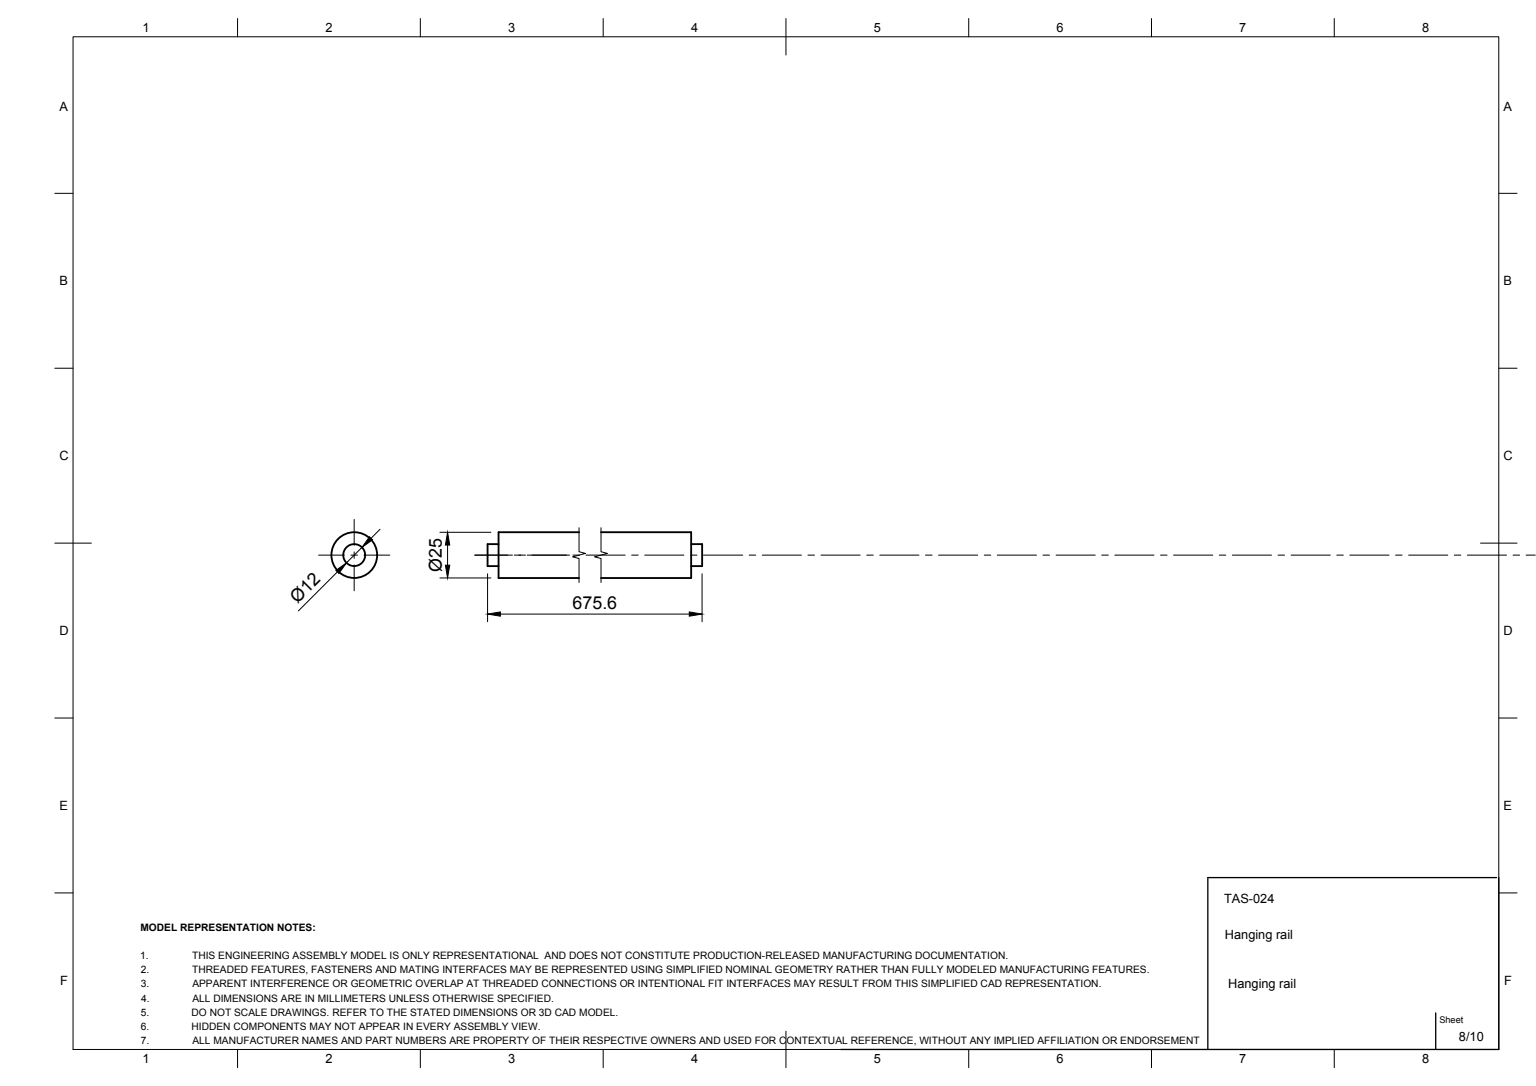
ISO-10303-21;
HEADER;
/* Generated by software containing ST-Developer
 * from STEP Tools, Inc. (www.steptools.com) 
 */

FILE_DESCRIPTION(
/* description */ (''),
/* implementation_level */ '2;1');

FILE_NAME(
/* name */ 'Hanging rail.step',
/* time_stamp */ '2026-11-15T17:53:25-08:00',
/* author */ (''),
/* organization */ (''),
/* preprocessor_version */ 'ST-DEVELOPER v20.2',
/* originating_system */ 'Autodesk Translation Framework v15.17.0.0',
/* authorisation */ '');

FILE_SCHEMA (('AUTOMOTIVE_DESIGN { 1 0 10303 214 3 1 1 }'));
ENDSEC;

DATA;
#10=MECHANICAL_DESIGN_GEOMETRIC_PRESENTATION_REPRESENTATION('',(#136),#2673);
#120=SHAPE_REPRESENTATION_RELATIONSHIP('SRR','None',#2728,#128);
#128=ADVANCED_BREP_SHAPE_REPRESENTATION('',(#144),#2670);
#136=STYLED_ITEM('',(#2777),#144);
#144=MANIFOLD_SOLID_BREP('Body1',#1522);
#157=FACE_BOUND('',#412,.T.);
#158=FACE_BOUND('',#414,.T.);
#224=PLANE('',#1718);
#225=PLANE('',#1722);
#226=PLANE('',#1726);
#227=PLANE('',#1727);
#307=FACE_OUTER_BOUND('',#406,.T.);
#308=FACE_OUTER_BOUND('',#407,.T.);
#309=FACE_OUTER_BOUND('',#408,.T.);
#310=FACE_OUTER_BOUND('',#409,.T.);
#311=FACE_OUTER_BOUND('',#410,.T.);
#312=FACE_OUTER_BOUND('',#411,.T.);
#313=FACE_OUTER_BOUND('',#413,.T.);
#406=EDGE_LOOP('',(#1376,#1377,#1378,#1379));
#407=EDGE_LOOP('',(#1380));
#408=EDGE_LOOP('',(#1381,#1382,#1383,#1384));
#409=EDGE_LOOP('',(#1385));
#410=EDGE_LOOP('',(#1386,#1387,#1388,#1389));
#411=EDGE_LOOP('',(#1390));
#412=EDGE_LOOP('',(#1391));
#413=EDGE_LOOP('',(#1392));
#414=EDGE_LOOP('',(#1393));
#566=LINE('',#2585,#714);
#567=LINE('',#2592,#715);
#568=LINE('',#2599,#716);
#714=VECTOR('',#2118,0.6);
#715=VECTOR('',#2127,0.6);
#716=VECTOR('',#2136,1.25);
#740=CIRCLE('',#1716,0.6);
#741=CIRCLE('',#1717,0.6);
#742=CIRCLE('',#1720,0.6);
#743=CIRCLE('',#1721,0.6);
#744=CIRCLE('',#1724,1.25);
#745=CIRCLE('',#1725,1.25);
#860=VERTEX_POINT('',#2582);
#861=VERTEX_POINT('',#2584);
#862=VERTEX_POINT('',#2589);
#863=VERTEX_POINT('',#2591);
#864=VERTEX_POINT('',#2596);
#865=VERTEX_POINT('',#2598);
#1034=EDGE_CURVE('',#860,#860,#740,.T.);
#1035=EDGE_CURVE('',#860,#861,#566,.T.);
#1036=EDGE_CURVE('',#861,#861,#741,.T.);
#1037=EDGE_CURVE('',#862,#862,#742,.T.);
#1038=EDGE_CURVE('',#862,#863,#567,.T.);
#1039=EDGE_CURVE('',#863,#863,#743,.T.);
#1040=EDGE_CURVE('',#864,#864,#744,.T.);
#1041=EDGE_CURVE('',#864,#865,#568,.T.);
#1042=EDGE_CURVE('',#865,#865,#745,.T.);
#1376=ORIENTED_EDGE('',*,*,#1034,.F.);
#1377=ORIENTED_EDGE('',*,*,#1035,.T.);
#1378=ORIENTED_EDGE('',*,*,#1036,.F.);
#1379=ORIENTED_EDGE('',*,*,#1035,.F.);
#1380=ORIENTED_EDGE('',*,*,#1034,.T.);
#1381=ORIENTED_EDGE('',*,*,#1037,.F.);
#1382=ORIENTED_EDGE('',*,*,#1038,.T.);
#1383=ORIENTED_EDGE('',*,*,#1039,.T.);
#1384=ORIENTED_EDGE('',*,*,#1038,.F.);
#1385=ORIENTED_EDGE('',*,*,#1039,.F.);
#1386=ORIENTED_EDGE('',*,*,#1040,.F.);
#1387=ORIENTED_EDGE('',*,*,#1041,.T.);
#1388=ORIENTED_EDGE('',*,*,#1042,.T.);
#1389=ORIENTED_EDGE('',*,*,#1041,.F.);
#1390=ORIENTED_EDGE('',*,*,#1040,.T.);
#1391=ORIENTED_EDGE('',*,*,#1036,.T.);
#1392=ORIENTED_EDGE('',*,*,#1042,.F.);
#1393=ORIENTED_EDGE('',*,*,#1037,.T.);
#1422=CYLINDRICAL_SURFACE('',#1715,0.6);
#1423=CYLINDRICAL_SURFACE('',#1719,0.6);
#1424=CYLINDRICAL_SURFACE('',#1723,1.25);
#1502=ADVANCED_FACE('',(#307),#1422,.T.);
#1503=ADVANCED_FACE('',(#308),#224,.T.);
#1504=ADVANCED_FACE('',(#309),#1423,.T.);
#1505=ADVANCED_FACE('',(#310),#225,.F.);
#1506=ADVANCED_FACE('',(#311),#1424,.T.);
#1507=ADVANCED_FACE('',(#312,#157),#226,.T.);
#1508=ADVANCED_FACE('',(#313,#158),#227,.F.);
#1522=CLOSED_SHELL('',(#1502,#1503,#1504,#1505,#1506,#1507,#1508));
#1714=AXIS2_PLACEMENT_3D('',#2580,#2112,#2113);
#1715=AXIS2_PLACEMENT_3D('',#2581,#2114,#2115);
#1716=AXIS2_PLACEMENT_3D('',#2583,#2116,#2117);
#1717=AXIS2_PLACEMENT_3D('',#2586,#2119,#2120);
#1718=AXIS2_PLACEMENT_3D('',#2587,#2121,#2122);
#1719=AXIS2_PLACEMENT_3D('',#2588,#2123,#2124);
#1720=AXIS2_PLACEMENT_3D('',#2590,#2125,#2126);
#1721=AXIS2_PLACEMENT_3D('',#2593,#2128,#2129);
#1722=AXIS2_PLACEMENT_3D('',#2594,#2130,#2131);
#1723=AXIS2_PLACEMENT_3D('',#2595,#2132,#2133);
#1724=AXIS2_PLACEMENT_3D('',#2597,#2134,#2135);
#1725=AXIS2_PLACEMENT_3D('',#2600,#2137,#2138);
#1726=AXIS2_PLACEMENT_3D('',#2601,#2139,#2140);
#1727=AXIS2_PLACEMENT_3D('',#2602,#2141,#2142);
#2112=DIRECTION('axis',(0.,0.,1.));
#2113=DIRECTION('refdir',(1.,0.,0.));
#2114=DIRECTION('center_axis',(0.,0.,1.));
#2115=DIRECTION('ref_axis',(1.,0.,0.));
#2116=DIRECTION('center_axis',(0.,0.,1.));
#2117=DIRECTION('ref_axis',(1.,0.,0.));
#2118=DIRECTION('',(0.,0.,-1.));
#2119=DIRECTION('center_axis',(0.,0.,-1.));
#2120=DIRECTION('ref_axis',(1.,0.,0.));
#2121=DIRECTION('center_axis',(0.,0.,1.));
#2122=DIRECTION('ref_axis',(1.,0.,0.));
#2123=DIRECTION('center_axis',(0.,0.,1.));
#2124=DIRECTION('ref_axis',(1.,0.,0.));
#2125=DIRECTION('center_axis',(0.,0.,1.));
#2126=DIRECTION('ref_axis',(1.,0.,0.));
#2127=DIRECTION('',(0.,0.,-1.));
#2128=DIRECTION('center_axis',(0.,0.,1.));
#2129=DIRECTION('ref_axis',(1.,0.,0.));
#2130=DIRECTION('center_axis',(0.,0.,1.));
#2131=DIRECTION('ref_axis',(1.,0.,0.));
#2132=DIRECTION('center_axis',(0.,0.,1.));
#2133=DIRECTION('ref_axis',(1.,0.,0.));
#2134=DIRECTION('center_axis',(0.,0.,1.));
#2135=DIRECTION('ref_axis',(1.,0.,0.));
#2136=DIRECTION('',(0.,0.,-1.));
#2137=DIRECTION('center_axis',(0.,0.,1.));
#2138=DIRECTION('ref_axis',(1.,0.,0.));
#2139=DIRECTION('center_axis',(0.,0.,1.));
#2140=DIRECTION('ref_axis',(1.,0.,0.));
#2141=DIRECTION('center_axis',(0.,0.,1.));
#2142=DIRECTION('ref_axis',(1.,0.,0.));
#2580=CARTESIAN_POINT('',(0.,0.,0.));
#2581=CARTESIAN_POINT('Origin',(0.,0.,66.36));
#2582=CARTESIAN_POINT('',(-0.6,-7.34788079488412E-17,66.96));
#2583=CARTESIAN_POINT('Origin',(0.,0.,66.96));
#2584=CARTESIAN_POINT('',(-0.6,-7.34788079488412E-17,66.36));
#2585=CARTESIAN_POINT('',(-0.6,-7.34788079488412E-17,66.36));
#2586=CARTESIAN_POINT('Origin',(0.,0.,66.36));
#2587=CARTESIAN_POINT('Origin',(0.,0.,66.96));
#2588=CARTESIAN_POINT('Origin',(0.,0.,-0.6));
#2589=CARTESIAN_POINT('',(-0.6,-7.34788079488412E-17,0.));
#2590=CARTESIAN_POINT('Origin',(0.,0.,0.));
#2591=CARTESIAN_POINT('',(-0.6,-7.34788079488412E-17,-0.6));
#2592=CARTESIAN_POINT('',(-0.6,-7.34788079488412E-17,-0.6));
#2593=CARTESIAN_POINT('Origin',(0.,0.,-0.6));
#2594=CARTESIAN_POINT('Origin',(0.,0.,-0.6));
#2595=CARTESIAN_POINT('Origin',(0.,0.,0.));
#2596=CARTESIAN_POINT('',(-1.25,-1.53080849893419E-16,66.36));
#2597=CARTESIAN_POINT('Origin',(0.,0.,66.36));
#2598=CARTESIAN_POINT('',(-1.25,-1.53080849893419E-16,0.));
#2599=CARTESIAN_POINT('',(-1.25,-1.53080849893419E-16,0.));
#2600=CARTESIAN_POINT('Origin',(0.,0.,0.));
#2601=CARTESIAN_POINT('Origin',(0.,0.,66.36));
#2602=CARTESIAN_POINT('Origin',(0.,0.,0.));
#2660=UNCERTAINTY_MEASURE_WITH_UNIT(LENGTH_MEASURE(0.001),#2674,
'DISTANCE_ACCURACY_VALUE',
'Maximum model space distance between geometric entities at asserted c
onnectivities');
#2663=UNCERTAINTY_MEASURE_WITH_UNIT(LENGTH_MEASURE(0.001),#2674,
'DISTANCE_ACCURACY_VALUE',
'Maximum model space distance between geometric entities at asserted c
onnectivities');
#2670=(
GEOMETRIC_REPRESENTATION_CONTEXT(3)
GLOBAL_UNCERTAINTY_ASSIGNED_CONTEXT((#2660))
GLOBAL_UNIT_ASSIGNED_CONTEXT((#2674,#2676,#2677))
REPRESENTATION_CONTEXT('','3D')
);
#2673=(
GEOMETRIC_REPRESENTATION_CONTEXT(3)
GLOBAL_UNCERTAINTY_ASSIGNED_CONTEXT((#2663))
GLOBAL_UNIT_ASSIGNED_CONTEXT((#2674,#2676,#2677))
REPRESENTATION_CONTEXT('','3D')
);
#2674=(
LENGTH_UNIT()
NAMED_UNIT(*)
SI_UNIT(.CENTI.,.METRE.)
);
#2676=(
NAMED_UNIT(*)
PLANE_ANGLE_UNIT()
SI_UNIT($,.RADIAN.)
);
#2677=(
NAMED_UNIT(*)
SI_UNIT($,.STERADIAN.)
SOLID_ANGLE_UNIT()
);
#2684=SHAPE_DEFINITION_REPRESENTATION(#2693,#2728);
#2693=PRODUCT_DEFINITION_SHAPE('',$,#2738);
#2728=SHAPE_REPRESENTATION('',(#1714),#2670);
#2731=PRODUCT_DEFINITION_CONTEXT('part definition',#2760,'design');
#2738=PRODUCT_DEFINITION('Hanging rail','Hanging rail',#2747,#2731);
#2747=PRODUCT_DEFINITION_FORMATION('',$,#2768);
#2760=APPLICATION_CONTEXT(
'Core Data for Automotive Mechanical Design Process');
#2761=PRODUCT_CONTEXT('part definition',#2760,'mechanical');
#2768=PRODUCT('Hanging rail','Hanging rail',$,(#2761));
#2777=PRESENTATION_STYLE_ASSIGNMENT((#2786));
#2786=SURFACE_STYLE_USAGE(.BOTH.,#2795);
#2795=SURFACE_SIDE_STYLE('',(#2804));
#2804=SURFACE_STYLE_FILL_AREA(#2813);
#2813=FILL_AREA_STYLE('Hanging rail finish',(#2822));
#2822=FILL_AREA_STYLE_COLOUR('Hanging rail finish',#2831);
#2831=COLOUR_RGB('Hanging rail finish',0.607843137254902,0.647058823529412,
0.701960784313725);
ENDSEC;
END-ISO-10303-21;
